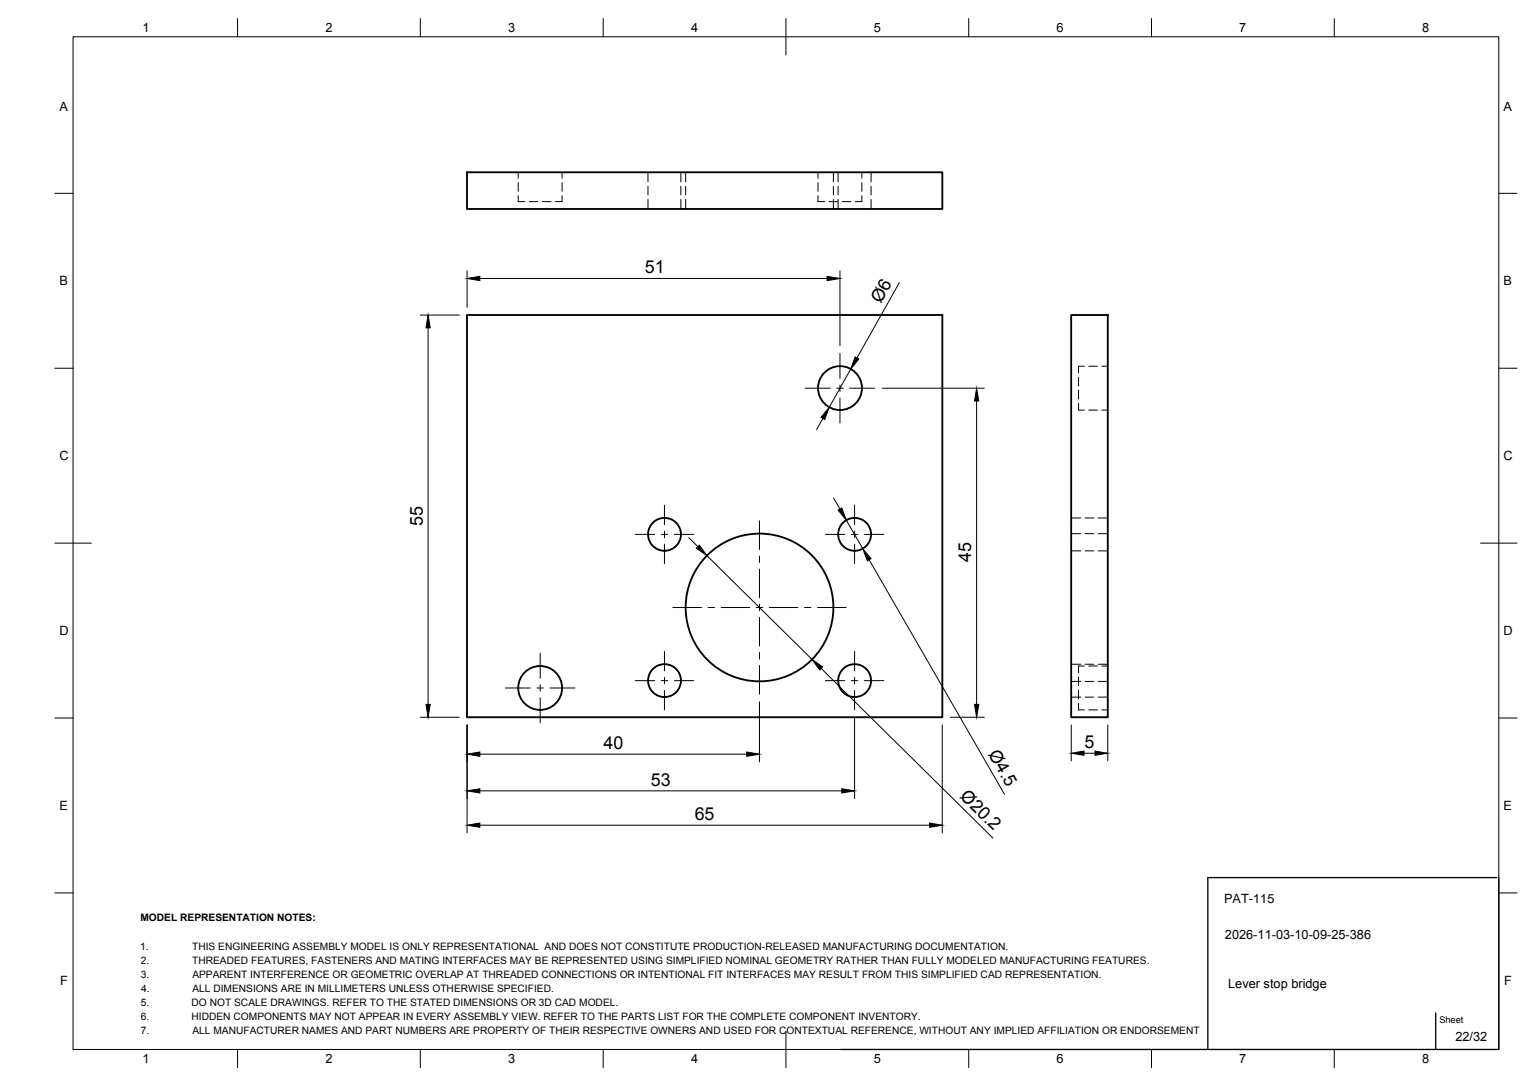
ISO-10303-21;
HEADER;
/* Generated by software containing ST-Developer
 * from STEP Tools, Inc. (www.steptools.com) 
 */

FILE_DESCRIPTION(
/* description */ ('Union bypass pipe loop'),
/* implementation_level */ '2;1');

FILE_NAME(
/* name */ 'Lever stop bridge.step',
/* time_stamp */ '2026-10-27T21:00:29-07:00',
/* author */ (''),
/* organization */ (''),
/* preprocessor_version */ 'ST-DEVELOPER v20.2',
/* originating_system */ 'Autodesk Translation Framework v15.17.0.0',
/* authorisation */ '');

FILE_SCHEMA (('AUTOMOTIVE_DESIGN { 1 0 10303 214 3 1 1 }'));
ENDSEC;

DATA;
#10=MECHANICAL_DESIGN_GEOMETRIC_PRESENTATION_REPRESENTATION('',(#451),#10095);
#387=SHAPE_REPRESENTATION_RELATIONSHIP('SRR','None',#10256,#419);
#419=ADVANCED_BREP_SHAPE_REPRESENTATION('',(#483),#10068);
#451=STYLED_ITEM('',(#10486),#483);
#483=MANIFOLD_SOLID_BREP('Body1',#5522);
#553=FACE_BOUND('',#1294,.T.);
#554=FACE_BOUND('',#1295,.T.);
#555=FACE_BOUND('',#1296,.T.);
#556=FACE_BOUND('',#1297,.T.);
#557=FACE_BOUND('',#1298,.T.);
#558=FACE_BOUND('',#1299,.T.);
#559=FACE_BOUND('',#1300,.T.);
#560=FACE_BOUND('',#1302,.T.);
#561=FACE_BOUND('',#1303,.T.);
#562=FACE_BOUND('',#1304,.T.);
#563=FACE_BOUND('',#1305,.T.);
#564=FACE_BOUND('',#1306,.T.);
#674=PLANE('',#6055);
#675=PLANE('',#6059);
#676=PLANE('',#6075);
#677=PLANE('',#6076);
#678=PLANE('',#6077);
#679=PLANE('',#6078);
#680=PLANE('',#6079);
#681=PLANE('',#6080);
#906=FACE_OUTER_BOUND('',#1280,.T.);
#907=FACE_OUTER_BOUND('',#1281,.T.);
#908=FACE_OUTER_BOUND('',#1282,.T.);
#909=FACE_OUTER_BOUND('',#1283,.T.);
#910=FACE_OUTER_BOUND('',#1284,.T.);
#911=FACE_OUTER_BOUND('',#1285,.T.);
#912=FACE_OUTER_BOUND('',#1286,.T.);
#913=FACE_OUTER_BOUND('',#1287,.T.);
#914=FACE_OUTER_BOUND('',#1288,.T.);
#915=FACE_OUTER_BOUND('',#1289,.T.);
#916=FACE_OUTER_BOUND('',#1290,.T.);
#917=FACE_OUTER_BOUND('',#1291,.T.);
#918=FACE_OUTER_BOUND('',#1292,.T.);
#919=FACE_OUTER_BOUND('',#1293,.T.);
#920=FACE_OUTER_BOUND('',#1301,.T.);
#1280=EDGE_LOOP('',(#4046,#4047,#4048,#4049));
#1281=EDGE_LOOP('',(#4050));
#1282=EDGE_LOOP('',(#4051,#4052,#4053,#4054));
#1283=EDGE_LOOP('',(#4055));
#1284=EDGE_LOOP('',(#4056,#4057,#4058,#4059));
#1285=EDGE_LOOP('',(#4060,#4061,#4062,#4063));
#1286=EDGE_LOOP('',(#4064,#4065,#4066,#4067));
#1287=EDGE_LOOP('',(#4068,#4069,#4070,#4071));
#1288=EDGE_LOOP('',(#4072,#4073,#4074,#4075));
#1289=EDGE_LOOP('',(#4076,#4077,#4078,#4079));
#1290=EDGE_LOOP('',(#4080,#4081,#4082,#4083));
#1291=EDGE_LOOP('',(#4084,#4085,#4086,#4087));
#1292=EDGE_LOOP('',(#4088,#4089,#4090,#4091));
#1293=EDGE_LOOP('',(#4092,#4093,#4094,#4095));
#1294=EDGE_LOOP('',(#4096));
#1295=EDGE_LOOP('',(#4097));
#1296=EDGE_LOOP('',(#4098));
#1297=EDGE_LOOP('',(#4099));
#1298=EDGE_LOOP('',(#4100));
#1299=EDGE_LOOP('',(#4101));
#1300=EDGE_LOOP('',(#4102));
#1301=EDGE_LOOP('',(#4103,#4104,#4105,#4106));
#1302=EDGE_LOOP('',(#4107));
#1303=EDGE_LOOP('',(#4108));
#1304=EDGE_LOOP('',(#4109));
#1305=EDGE_LOOP('',(#4110));
#1306=EDGE_LOOP('',(#4111));
#1711=LINE('',#8765,#2087);
#1712=LINE('',#8772,#2088);
#1713=LINE('',#8779,#2089);
#1714=LINE('',#8785,#2090);
#1715=LINE('',#8791,#2091);
#1716=LINE('',#8797,#2092);
#1717=LINE('',#8803,#2093);
#1718=LINE('',#8808,#2094);
#1719=LINE('',#8810,#2095);
#1720=LINE('',#8812,#2096);
#1721=LINE('',#8813,#2097);
#1722=LINE('',#8816,#2098);
#1723=LINE('',#8818,#2099);
#1724=LINE('',#8819,#2100);
#1725=LINE('',#8822,#2101);
#1726=LINE('',#8824,#2102);
#1727=LINE('',#8825,#2103);
#1728=LINE('',#8827,#2104);
#1729=LINE('',#8828,#2105);
#2087=VECTOR('',#7005,0.3);
#2088=VECTOR('',#7014,0.3);
#2089=VECTOR('',#7023,0.225);
#2090=VECTOR('',#7030,0.225);
#2091=VECTOR('',#7037,0.225);
#2092=VECTOR('',#7044,0.225);
#2093=VECTOR('',#7051,1.01);
#2094=VECTOR('',#7056,1.);
#2095=VECTOR('',#7057,1.);
#2096=VECTOR('',#7058,1.);
#2097=VECTOR('',#7059,1.);
#2098=VECTOR('',#7062,1.);
#2099=VECTOR('',#7063,1.);
#2100=VECTOR('',#7064,1.);
#2101=VECTOR('',#7067,1.);
#2102=VECTOR('',#7068,1.);
#2103=VECTOR('',#7069,1.);
#2104=VECTOR('',#7072,1.);
#2105=VECTOR('',#7073,1.);
#2441=CIRCLE('',#6053,0.3);
#2442=CIRCLE('',#6054,0.3);
#2443=CIRCLE('',#6057,0.3);
#2444=CIRCLE('',#6058,0.3);
#2445=CIRCLE('',#6061,0.225);
#2446=CIRCLE('',#6062,0.225);
#2447=CIRCLE('',#6064,0.225);
#2448=CIRCLE('',#6065,0.225);
#2449=CIRCLE('',#6067,0.225);
#2450=CIRCLE('',#6068,0.225);
#2451=CIRCLE('',#6070,0.225);
#2452=CIRCLE('',#6071,0.225);
#2453=CIRCLE('',#6073,1.01);
#2454=CIRCLE('',#6074,1.01);
#2733=VERTEX_POINT('',#8762);
#2734=VERTEX_POINT('',#8764);
#2735=VERTEX_POINT('',#8769);
#2736=VERTEX_POINT('',#8771);
#2737=VERTEX_POINT('',#8776);
#2738=VERTEX_POINT('',#8778);
#2739=VERTEX_POINT('',#8782);
#2740=VERTEX_POINT('',#8784);
#2741=VERTEX_POINT('',#8788);
#2742=VERTEX_POINT('',#8790);
#2743=VERTEX_POINT('',#8794);
#2744=VERTEX_POINT('',#8796);
#2745=VERTEX_POINT('',#8800);
#2746=VERTEX_POINT('',#8802);
#2747=VERTEX_POINT('',#8806);
#2748=VERTEX_POINT('',#8807);
#2749=VERTEX_POINT('',#8809);
#2750=VERTEX_POINT('',#8811);
#2751=VERTEX_POINT('',#8815);
#2752=VERTEX_POINT('',#8817);
#2753=VERTEX_POINT('',#8821);
#2754=VERTEX_POINT('',#8823);
#3221=EDGE_CURVE('',#2733,#2733,#2441,.T.);
#3222=EDGE_CURVE('',#2733,#2734,#1711,.T.);
#3223=EDGE_CURVE('',#2734,#2734,#2442,.T.);
#3224=EDGE_CURVE('',#2735,#2735,#2443,.T.);
#3225=EDGE_CURVE('',#2735,#2736,#1712,.T.);
#3226=EDGE_CURVE('',#2736,#2736,#2444,.T.);
#3227=EDGE_CURVE('',#2737,#2737,#2445,.T.);
#3228=EDGE_CURVE('',#2737,#2738,#1713,.T.);
#3229=EDGE_CURVE('',#2738,#2738,#2446,.T.);
#3230=EDGE_CURVE('',#2739,#2739,#2447,.T.);
#3231=EDGE_CURVE('',#2739,#2740,#1714,.T.);
#3232=EDGE_CURVE('',#2740,#2740,#2448,.T.);
#3233=EDGE_CURVE('',#2741,#2741,#2449,.T.);
#3234=EDGE_CURVE('',#2741,#2742,#1715,.T.);
#3235=EDGE_CURVE('',#2742,#2742,#2450,.T.);
#3236=EDGE_CURVE('',#2743,#2743,#2451,.T.);
#3237=EDGE_CURVE('',#2743,#2744,#1716,.T.);
#3238=EDGE_CURVE('',#2744,#2744,#2452,.T.);
#3239=EDGE_CURVE('',#2745,#2745,#2453,.T.);
#3240=EDGE_CURVE('',#2745,#2746,#1717,.T.);
#3241=EDGE_CURVE('',#2746,#2746,#2454,.T.);
#3242=EDGE_CURVE('',#2747,#2748,#1718,.T.);
#3243=EDGE_CURVE('',#2748,#2749,#1719,.T.);
#3244=EDGE_CURVE('',#2750,#2749,#1720,.T.);
#3245=EDGE_CURVE('',#2747,#2750,#1721,.T.);
#3246=EDGE_CURVE('',#2751,#2747,#1722,.T.);
#3247=EDGE_CURVE('',#2752,#2750,#1723,.T.);
#3248=EDGE_CURVE('',#2751,#2752,#1724,.T.);
#3249=EDGE_CURVE('',#2753,#2751,#1725,.T.);
#3250=EDGE_CURVE('',#2754,#2752,#1726,.T.);
#3251=EDGE_CURVE('',#2753,#2754,#1727,.T.);
#3252=EDGE_CURVE('',#2748,#2753,#1728,.T.);
#3253=EDGE_CURVE('',#2749,#2754,#1729,.T.);
#4046=ORIENTED_EDGE('',*,*,#3221,.F.);
#4047=ORIENTED_EDGE('',*,*,#3222,.T.);
#4048=ORIENTED_EDGE('',*,*,#3223,.F.);
#4049=ORIENTED_EDGE('',*,*,#3222,.F.);
#4050=ORIENTED_EDGE('',*,*,#3221,.T.);
#4051=ORIENTED_EDGE('',*,*,#3224,.F.);
#4052=ORIENTED_EDGE('',*,*,#3225,.T.);
#4053=ORIENTED_EDGE('',*,*,#3226,.F.);
#4054=ORIENTED_EDGE('',*,*,#3225,.F.);
#4055=ORIENTED_EDGE('',*,*,#3224,.T.);
#4056=ORIENTED_EDGE('',*,*,#3227,.F.);
#4057=ORIENTED_EDGE('',*,*,#3228,.T.);
#4058=ORIENTED_EDGE('',*,*,#3229,.F.);
#4059=ORIENTED_EDGE('',*,*,#3228,.F.);
#4060=ORIENTED_EDGE('',*,*,#3230,.F.);
#4061=ORIENTED_EDGE('',*,*,#3231,.T.);
#4062=ORIENTED_EDGE('',*,*,#3232,.F.);
#4063=ORIENTED_EDGE('',*,*,#3231,.F.);
#4064=ORIENTED_EDGE('',*,*,#3233,.F.);
#4065=ORIENTED_EDGE('',*,*,#3234,.T.);
#4066=ORIENTED_EDGE('',*,*,#3235,.F.);
#4067=ORIENTED_EDGE('',*,*,#3234,.F.);
#4068=ORIENTED_EDGE('',*,*,#3236,.F.);
#4069=ORIENTED_EDGE('',*,*,#3237,.T.);
#4070=ORIENTED_EDGE('',*,*,#3238,.F.);
#4071=ORIENTED_EDGE('',*,*,#3237,.F.);
#4072=ORIENTED_EDGE('',*,*,#3239,.F.);
#4073=ORIENTED_EDGE('',*,*,#3240,.T.);
#4074=ORIENTED_EDGE('',*,*,#3241,.F.);
#4075=ORIENTED_EDGE('',*,*,#3240,.F.);
#4076=ORIENTED_EDGE('',*,*,#3242,.T.);
#4077=ORIENTED_EDGE('',*,*,#3243,.T.);
#4078=ORIENTED_EDGE('',*,*,#3244,.F.);
#4079=ORIENTED_EDGE('',*,*,#3245,.F.);
#4080=ORIENTED_EDGE('',*,*,#3246,.T.);
#4081=ORIENTED_EDGE('',*,*,#3245,.T.);
#4082=ORIENTED_EDGE('',*,*,#3247,.F.);
#4083=ORIENTED_EDGE('',*,*,#3248,.F.);
#4084=ORIENTED_EDGE('',*,*,#3249,.T.);
#4085=ORIENTED_EDGE('',*,*,#3248,.T.);
#4086=ORIENTED_EDGE('',*,*,#3250,.F.);
#4087=ORIENTED_EDGE('',*,*,#3251,.F.);
#4088=ORIENTED_EDGE('',*,*,#3252,.T.);
#4089=ORIENTED_EDGE('',*,*,#3251,.T.);
#4090=ORIENTED_EDGE('',*,*,#3253,.F.);
#4091=ORIENTED_EDGE('',*,*,#3243,.F.);
#4092=ORIENTED_EDGE('',*,*,#3253,.T.);
#4093=ORIENTED_EDGE('',*,*,#3250,.T.);
#4094=ORIENTED_EDGE('',*,*,#3247,.T.);
#4095=ORIENTED_EDGE('',*,*,#3244,.T.);
#4096=ORIENTED_EDGE('',*,*,#3223,.T.);
#4097=ORIENTED_EDGE('',*,*,#3226,.T.);
#4098=ORIENTED_EDGE('',*,*,#3241,.T.);
#4099=ORIENTED_EDGE('',*,*,#3238,.T.);
#4100=ORIENTED_EDGE('',*,*,#3235,.T.);
#4101=ORIENTED_EDGE('',*,*,#3232,.T.);
#4102=ORIENTED_EDGE('',*,*,#3229,.T.);
#4103=ORIENTED_EDGE('',*,*,#3252,.F.);
#4104=ORIENTED_EDGE('',*,*,#3242,.F.);
#4105=ORIENTED_EDGE('',*,*,#3246,.F.);
#4106=ORIENTED_EDGE('',*,*,#3249,.F.);
#4107=ORIENTED_EDGE('',*,*,#3239,.T.);
#4108=ORIENTED_EDGE('',*,*,#3236,.T.);
#4109=ORIENTED_EDGE('',*,*,#3233,.T.);
#4110=ORIENTED_EDGE('',*,*,#3230,.T.);
#4111=ORIENTED_EDGE('',*,*,#3227,.T.);
#5109=CYLINDRICAL_SURFACE('',#6052,0.3);
#5110=CYLINDRICAL_SURFACE('',#6056,0.3);
#5111=CYLINDRICAL_SURFACE('',#6060,0.225);
#5112=CYLINDRICAL_SURFACE('',#6063,0.225);
#5113=CYLINDRICAL_SURFACE('',#6066,0.225);
#5114=CYLINDRICAL_SURFACE('',#6069,0.225);
#5115=CYLINDRICAL_SURFACE('',#6072,1.01);
#5255=ADVANCED_FACE('',(#906),#5109,.F.);
#5256=ADVANCED_FACE('',(#907),#674,.T.);
#5257=ADVANCED_FACE('',(#908),#5110,.F.);
#5258=ADVANCED_FACE('',(#909),#675,.T.);
#5259=ADVANCED_FACE('',(#910),#5111,.F.);
#5260=ADVANCED_FACE('',(#911),#5112,.F.);
#5261=ADVANCED_FACE('',(#912),#5113,.F.);
#5262=ADVANCED_FACE('',(#913),#5114,.F.);
#5263=ADVANCED_FACE('',(#914),#5115,.F.);
#5264=ADVANCED_FACE('',(#915),#676,.T.);
#5265=ADVANCED_FACE('',(#916),#677,.T.);
#5266=ADVANCED_FACE('',(#917),#678,.T.);
#5267=ADVANCED_FACE('',(#918),#679,.T.);
#5268=ADVANCED_FACE('',(#919,#553,#554,#555,#556,#557,#558,#559),#680,.T.);
#5269=ADVANCED_FACE('',(#920,#560,#561,#562,#563,#564),#681,.F.);
#5522=CLOSED_SHELL('',(#5255,#5256,#5257,#5258,#5259,#5260,#5261,#5262,
#5263,#5264,#5265,#5266,#5267,#5268,#5269));
#6051=AXIS2_PLACEMENT_3D('',#8760,#6999,#7000);
#6052=AXIS2_PLACEMENT_3D('',#8761,#7001,#7002);
#6053=AXIS2_PLACEMENT_3D('',#8763,#7003,#7004);
#6054=AXIS2_PLACEMENT_3D('',#8766,#7006,#7007);
#6055=AXIS2_PLACEMENT_3D('',#8767,#7008,#7009);
#6056=AXIS2_PLACEMENT_3D('',#8768,#7010,#7011);
#6057=AXIS2_PLACEMENT_3D('',#8770,#7012,#7013);
#6058=AXIS2_PLACEMENT_3D('',#8773,#7015,#7016);
#6059=AXIS2_PLACEMENT_3D('',#8774,#7017,#7018);
#6060=AXIS2_PLACEMENT_3D('',#8775,#7019,#7020);
#6061=AXIS2_PLACEMENT_3D('',#8777,#7021,#7022);
#6062=AXIS2_PLACEMENT_3D('',#8780,#7024,#7025);
#6063=AXIS2_PLACEMENT_3D('',#8781,#7026,#7027);
#6064=AXIS2_PLACEMENT_3D('',#8783,#7028,#7029);
#6065=AXIS2_PLACEMENT_3D('',#8786,#7031,#7032);
#6066=AXIS2_PLACEMENT_3D('',#8787,#7033,#7034);
#6067=AXIS2_PLACEMENT_3D('',#8789,#7035,#7036);
#6068=AXIS2_PLACEMENT_3D('',#8792,#7038,#7039);
#6069=AXIS2_PLACEMENT_3D('',#8793,#7040,#7041);
#6070=AXIS2_PLACEMENT_3D('',#8795,#7042,#7043);
#6071=AXIS2_PLACEMENT_3D('',#8798,#7045,#7046);
#6072=AXIS2_PLACEMENT_3D('',#8799,#7047,#7048);
#6073=AXIS2_PLACEMENT_3D('',#8801,#7049,#7050);
#6074=AXIS2_PLACEMENT_3D('',#8804,#7052,#7053);
#6075=AXIS2_PLACEMENT_3D('',#8805,#7054,#7055);
#6076=AXIS2_PLACEMENT_3D('',#8814,#7060,#7061);
#6077=AXIS2_PLACEMENT_3D('',#8820,#7065,#7066);
#6078=AXIS2_PLACEMENT_3D('',#8826,#7070,#7071);
#6079=AXIS2_PLACEMENT_3D('',#8829,#7074,#7075);
#6080=AXIS2_PLACEMENT_3D('',#8830,#7076,#7077);
#6999=DIRECTION('axis',(0.,0.,1.));
#7000=DIRECTION('refdir',(1.,0.,0.));
#7001=DIRECTION('center_axis',(0.,0.,1.));
#7002=DIRECTION('ref_axis',(1.,0.,0.));
#7003=DIRECTION('center_axis',(0.,0.,1.));
#7004=DIRECTION('ref_axis',(1.,0.,0.));
#7005=DIRECTION('',(0.,0.,1.));
#7006=DIRECTION('center_axis',(0.,0.,-1.));
#7007=DIRECTION('ref_axis',(1.,0.,0.));
#7008=DIRECTION('center_axis',(0.,0.,1.));
#7009=DIRECTION('ref_axis',(1.,0.,0.));
#7010=DIRECTION('center_axis',(0.,0.,1.));
#7011=DIRECTION('ref_axis',(1.,0.,0.));
#7012=DIRECTION('center_axis',(0.,0.,1.));
#7013=DIRECTION('ref_axis',(1.,0.,0.));
#7014=DIRECTION('',(0.,0.,1.));
#7015=DIRECTION('center_axis',(0.,0.,-1.));
#7016=DIRECTION('ref_axis',(1.,0.,0.));
#7017=DIRECTION('center_axis',(0.,0.,1.));
#7018=DIRECTION('ref_axis',(1.,0.,0.));
#7019=DIRECTION('center_axis',(0.,0.,1.));
#7020=DIRECTION('ref_axis',(1.,0.,0.));
#7021=DIRECTION('center_axis',(0.,0.,1.));
#7022=DIRECTION('ref_axis',(1.,0.,0.));
#7023=DIRECTION('',(0.,0.,1.));
#7024=DIRECTION('center_axis',(0.,0.,-1.));
#7025=DIRECTION('ref_axis',(1.,0.,0.));
#7026=DIRECTION('center_axis',(0.,0.,1.));
#7027=DIRECTION('ref_axis',(1.,0.,0.));
#7028=DIRECTION('center_axis',(0.,0.,1.));
#7029=DIRECTION('ref_axis',(1.,0.,0.));
#7030=DIRECTION('',(0.,0.,1.));
#7031=DIRECTION('center_axis',(0.,0.,-1.));
#7032=DIRECTION('ref_axis',(1.,0.,0.));
#7033=DIRECTION('center_axis',(0.,0.,1.));
#7034=DIRECTION('ref_axis',(1.,0.,0.));
#7035=DIRECTION('center_axis',(0.,0.,1.));
#7036=DIRECTION('ref_axis',(1.,0.,0.));
#7037=DIRECTION('',(0.,0.,1.));
#7038=DIRECTION('center_axis',(0.,0.,-1.));
#7039=DIRECTION('ref_axis',(1.,0.,0.));
#7040=DIRECTION('center_axis',(0.,0.,1.));
#7041=DIRECTION('ref_axis',(1.,0.,0.));
#7042=DIRECTION('center_axis',(0.,0.,1.));
#7043=DIRECTION('ref_axis',(1.,0.,0.));
#7044=DIRECTION('',(0.,0.,1.));
#7045=DIRECTION('center_axis',(0.,0.,-1.));
#7046=DIRECTION('ref_axis',(1.,0.,0.));
#7047=DIRECTION('center_axis',(0.,0.,1.));
#7048=DIRECTION('ref_axis',(1.,0.,0.));
#7049=DIRECTION('center_axis',(0.,0.,1.));
#7050=DIRECTION('ref_axis',(1.,0.,0.));
#7051=DIRECTION('',(0.,0.,1.));
#7052=DIRECTION('center_axis',(0.,0.,-1.));
#7053=DIRECTION('ref_axis',(1.,0.,0.));
#7054=DIRECTION('center_axis',(0.,1.,0.));
#7055=DIRECTION('ref_axis',(-1.,0.,0.));
#7056=DIRECTION('',(-1.,0.,0.));
#7057=DIRECTION('',(0.,0.,1.));
#7058=DIRECTION('',(-1.,0.,0.));
#7059=DIRECTION('',(0.,0.,1.));
#7060=DIRECTION('center_axis',(1.,0.,0.));
#7061=DIRECTION('ref_axis',(0.,1.,0.));
#7062=DIRECTION('',(0.,1.,0.));
#7063=DIRECTION('',(0.,1.,0.));
#7064=DIRECTION('',(0.,0.,1.));
#7065=DIRECTION('center_axis',(0.,-1.,0.));
#7066=DIRECTION('ref_axis',(1.,0.,0.));
#7067=DIRECTION('',(1.,0.,0.));
#7068=DIRECTION('',(1.,0.,0.));
#7069=DIRECTION('',(0.,0.,1.));
#7070=DIRECTION('center_axis',(-1.,0.,0.));
#7071=DIRECTION('ref_axis',(0.,-1.,0.));
#7072=DIRECTION('',(0.,-1.,0.));
#7073=DIRECTION('',(0.,-1.,0.));
#7074=DIRECTION('center_axis',(0.,0.,1.));
#7075=DIRECTION('ref_axis',(1.,0.,0.));
#7076=DIRECTION('center_axis',(0.,0.,1.));
#7077=DIRECTION('ref_axis',(1.,0.,0.));
#8760=CARTESIAN_POINT('',(0.,0.,0.));
#8761=CARTESIAN_POINT('Origin',(-1.1,-3.,8.1));
#8762=CARTESIAN_POINT('',(-1.4,-3.,8.1));
#8763=CARTESIAN_POINT('Origin',(-1.1,-3.,8.1));
#8764=CARTESIAN_POINT('',(-1.4,-3.,8.5));
#8765=CARTESIAN_POINT('',(-1.4,-3.,8.1));
#8766=CARTESIAN_POINT('Origin',(-1.1,-3.,8.5));
#8767=CARTESIAN_POINT('Origin',(-1.1,-3.,8.1));
#8768=CARTESIAN_POINT('Origin',(3.,1.1,8.1));
#8769=CARTESIAN_POINT('',(2.7,1.1,8.1));
#8770=CARTESIAN_POINT('Origin',(3.,1.1,8.1));
#8771=CARTESIAN_POINT('',(2.7,1.1,8.5));
#8772=CARTESIAN_POINT('',(2.7,1.1,8.1));
#8773=CARTESIAN_POINT('Origin',(3.,1.1,8.5));
#8774=CARTESIAN_POINT('Origin',(3.,1.1,8.1));
#8775=CARTESIAN_POINT('Origin',(1.3,-1.,7.9));
#8776=CARTESIAN_POINT('',(1.075,-1.,8.));
#8777=CARTESIAN_POINT('Origin',(1.3,-1.,8.));
#8778=CARTESIAN_POINT('',(1.075,-1.,8.5));
#8779=CARTESIAN_POINT('',(1.075,-1.,7.9));
#8780=CARTESIAN_POINT('Origin',(1.3,-1.,8.5));
#8781=CARTESIAN_POINT('Origin',(-1.3,1.,7.9));
#8782=CARTESIAN_POINT('',(-1.525,1.,8.));
#8783=CARTESIAN_POINT('Origin',(-1.3,1.,8.));
#8784=CARTESIAN_POINT('',(-1.525,1.,8.5));
#8785=CARTESIAN_POINT('',(-1.525,1.,7.9));
#8786=CARTESIAN_POINT('Origin',(-1.3,1.,8.5));
#8787=CARTESIAN_POINT('Origin',(-1.3,-1.,7.9));
#8788=CARTESIAN_POINT('',(-1.525,-1.,8.));
#8789=CARTESIAN_POINT('Origin',(-1.3,-1.,8.));
#8790=CARTESIAN_POINT('',(-1.525,-1.,8.5));
#8791=CARTESIAN_POINT('',(-1.525,-1.,7.9));
#8792=CARTESIAN_POINT('Origin',(-1.3,-1.,8.5));
#8793=CARTESIAN_POINT('Origin',(1.3,1.,7.9));
#8794=CARTESIAN_POINT('',(1.075,1.,8.));
#8795=CARTESIAN_POINT('Origin',(1.3,1.,8.));
#8796=CARTESIAN_POINT('',(1.075,1.,8.5));
#8797=CARTESIAN_POINT('',(1.075,1.,7.9));
#8798=CARTESIAN_POINT('Origin',(1.3,1.,8.5));
#8799=CARTESIAN_POINT('Origin',(0.,0.,7.9));
#8800=CARTESIAN_POINT('',(-1.01,-1.23689326713883E-16,8.));
#8801=CARTESIAN_POINT('Origin',(0.,0.,8.));
#8802=CARTESIAN_POINT('',(-1.01,1.23689326713883E-16,8.5));
#8803=CARTESIAN_POINT('',(-1.01,-1.23689326713883E-16,7.9));
#8804=CARTESIAN_POINT('Origin',(0.,0.,8.5));
#8805=CARTESIAN_POINT('Origin',(4.,1.5,8.));
#8806=CARTESIAN_POINT('',(4.,1.5,8.));
#8807=CARTESIAN_POINT('',(-2.5,1.5,8.));
#8808=CARTESIAN_POINT('',(4.,1.5,8.));
#8809=CARTESIAN_POINT('',(-2.5,1.5,8.5));
#8810=CARTESIAN_POINT('',(-2.5,1.5,8.));
#8811=CARTESIAN_POINT('',(4.,1.5,8.5));
#8812=CARTESIAN_POINT('',(4.,1.5,8.5));
#8813=CARTESIAN_POINT('',(4.,1.5,8.));
#8814=CARTESIAN_POINT('Origin',(4.,-4.,8.));
#8815=CARTESIAN_POINT('',(4.,-4.,8.));
#8816=CARTESIAN_POINT('',(4.,-4.,8.));
#8817=CARTESIAN_POINT('',(4.,-4.,8.5));
#8818=CARTESIAN_POINT('',(4.,-4.,8.5));
#8819=CARTESIAN_POINT('',(4.,-4.,8.));
#8820=CARTESIAN_POINT('Origin',(-2.5,-4.,8.));
#8821=CARTESIAN_POINT('',(-2.5,-4.,8.));
#8822=CARTESIAN_POINT('',(-2.5,-4.,8.));
#8823=CARTESIAN_POINT('',(-2.5,-4.,8.5));
#8824=CARTESIAN_POINT('',(-2.5,-4.,8.5));
#8825=CARTESIAN_POINT('',(-2.5,-4.,8.));
#8826=CARTESIAN_POINT('Origin',(-2.5,1.5,8.));
#8827=CARTESIAN_POINT('',(-2.5,1.5,8.));
#8828=CARTESIAN_POINT('',(-2.5,1.5,8.5));
#8829=CARTESIAN_POINT('Origin',(0.75,-1.25,8.5));
#8830=CARTESIAN_POINT('Origin',(0.75,-1.25,8.));
#10031=UNCERTAINTY_MEASURE_WITH_UNIT(LENGTH_MEASURE(0.001),#10096,
'DISTANCE_ACCURACY_VALUE',
'Maximum model space distance between geometric entities at asserted c
onnectivities');
#10058=UNCERTAINTY_MEASURE_WITH_UNIT(LENGTH_MEASURE(0.001),#10096,
'DISTANCE_ACCURACY_VALUE',
'Maximum model space distance between geometric entities at asserted c
onnectivities');
#10068=(
GEOMETRIC_REPRESENTATION_CONTEXT(3)
GLOBAL_UNCERTAINTY_ASSIGNED_CONTEXT((#10031))
GLOBAL_UNIT_ASSIGNED_CONTEXT((#10096,#10098,#10099))
REPRESENTATION_CONTEXT('','3D')
);
#10095=(
GEOMETRIC_REPRESENTATION_CONTEXT(3)
GLOBAL_UNCERTAINTY_ASSIGNED_CONTEXT((#10058))
GLOBAL_UNIT_ASSIGNED_CONTEXT((#10096,#10098,#10099))
REPRESENTATION_CONTEXT('','3D')
);
#10096=(
LENGTH_UNIT()
NAMED_UNIT(*)
SI_UNIT(.CENTI.,.METRE.)
);
#10098=(
NAMED_UNIT(*)
PLANE_ANGLE_UNIT()
SI_UNIT($,.RADIAN.)
);
#10099=(
NAMED_UNIT(*)
SI_UNIT($,.STERADIAN.)
SOLID_ANGLE_UNIT()
);
#10109=SHAPE_DEFINITION_REPRESENTATION(#10145,#10256);
#10145=PRODUCT_DEFINITION_SHAPE('',$,#10293);
#10256=SHAPE_REPRESENTATION('',(#6051),#10068);
#10283=PRODUCT_DEFINITION_CONTEXT('part definition',#10393,'design');
#10293=PRODUCT_DEFINITION('Lever stop bridge','Lever stop bridge',#10329,
#10283);
#10329=PRODUCT_DEFINITION_FORMATION('',$,#10404);
#10393=APPLICATION_CONTEXT(
'Core Data for Automotive Mechanical Design Process');
#10394=PRODUCT_CONTEXT('part definition',#10393,'mechanical');
#10404=PRODUCT('Lever stop bridge','Lever stop bridge',
'Lever stop bridge',(#10394));
#10480=COLOUR_RGB('Light Blue',0.38,0.62,0.78);
#10481=FILL_AREA_STYLE_COLOUR('',#10480);
#10482=FILL_AREA_STYLE('',(#10481));
#10483=SURFACE_STYLE_FILL_AREA(#10482);
#10484=SURFACE_SIDE_STYLE('',(#10483));
#10485=SURFACE_STYLE_USAGE(.BOTH.,#10484);
#10486=PRESENTATION_STYLE_ASSIGNMENT((#10485));
ENDSEC;
END-ISO-10303-21;
